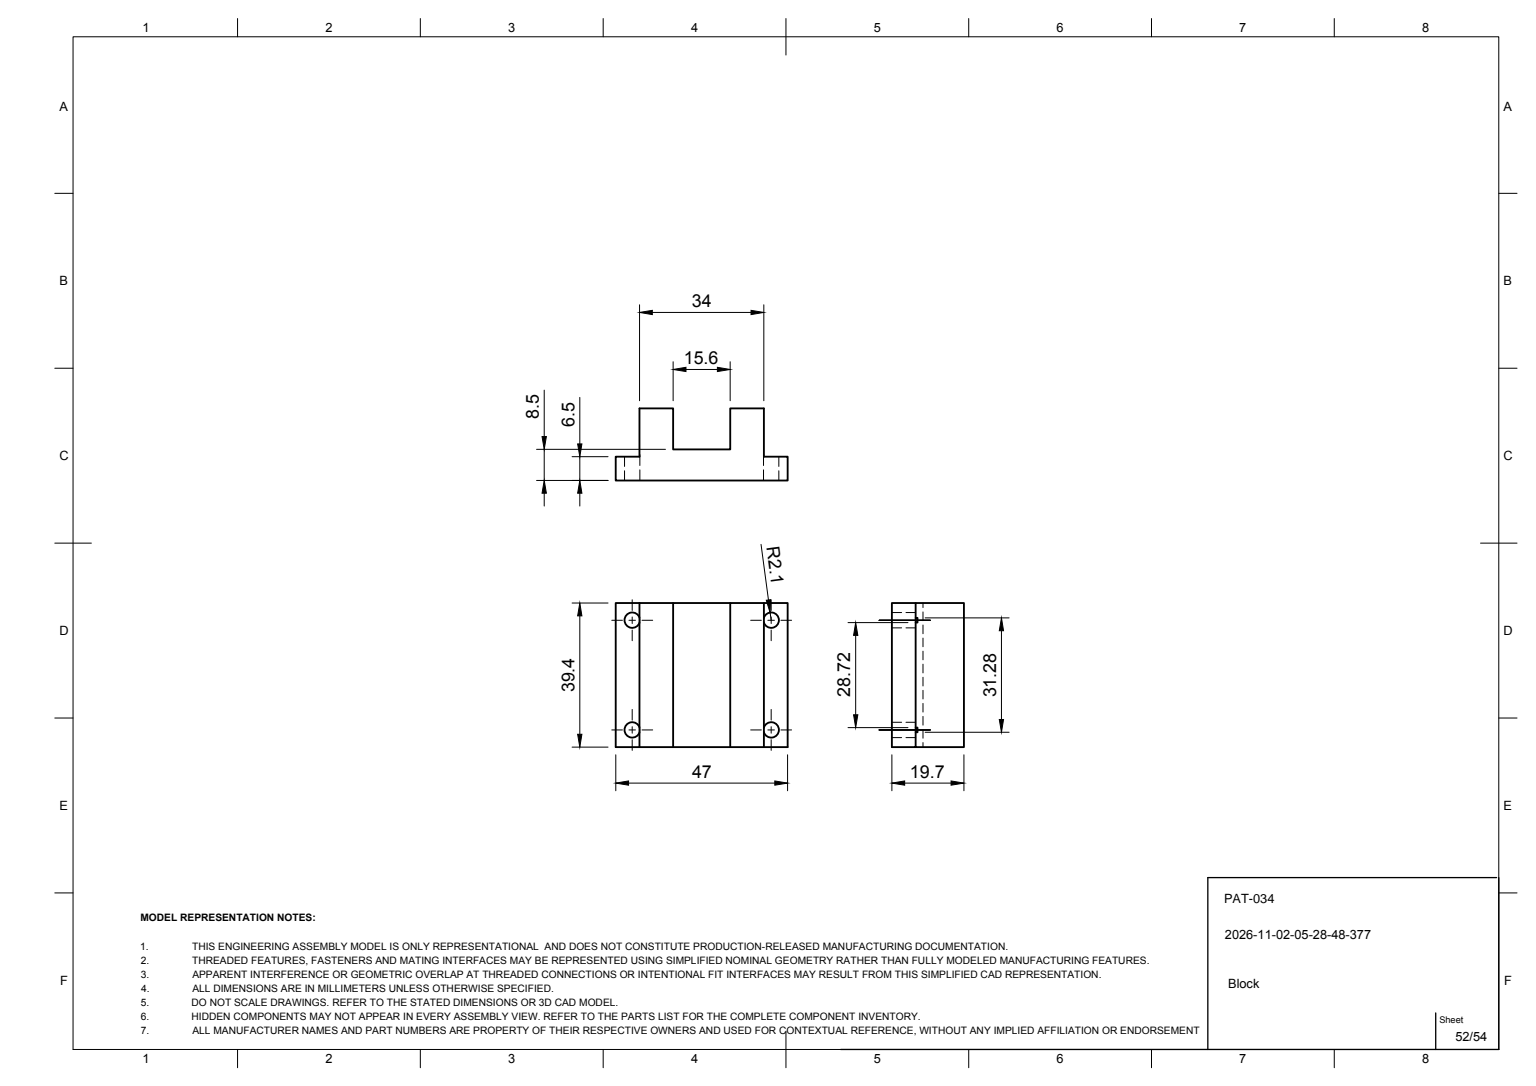
ISO-10303-21;
HEADER;
/* Generated by software containing ST-Developer
 * from STEP Tools, Inc. (www.steptools.com) 
 */

FILE_DESCRIPTION(
/* description */ ('Fatigue rig crank-slider'),
/* implementation_level */ '2;1');

FILE_NAME(
/* name */ 'Block.step',
/* time_stamp */ '2026-10-28T03:24:50-07:00',
/* author */ (''),
/* organization */ (''),
/* preprocessor_version */ 'ST-DEVELOPER v20.2',
/* originating_system */ 'Autodesk Translation Framework v15.17.0.0',
/* authorisation */ '');

FILE_SCHEMA (('AUTOMOTIVE_DESIGN { 1 0 10303 214 3 1 1 }'));
ENDSEC;

DATA;
#10=MECHANICAL_DESIGN_GEOMETRIC_PRESENTATION_REPRESENTATION('',(#639),#16911);
#530=SHAPE_REPRESENTATION_RELATIONSHIP('SRR','None',#17175,#580);
#580=ADVANCED_BREP_SHAPE_REPRESENTATION('',(#696),#16904);
#639=STYLED_ITEM('',(#17466),#696);
#696=MANIFOLD_SOLID_BREP('Body1',#8932);
#888=FACE_BOUND('',#2369,.T.);
#889=FACE_BOUND('',#2370,.T.);
#890=FACE_BOUND('',#2371,.T.);
#891=FACE_BOUND('',#2372,.T.);
#1144=PLANE('',#10343);
#1145=PLANE('',#10349);
#1146=PLANE('',#10355);
#1147=PLANE('',#10361);
#1148=PLANE('',#10367);
#1149=PLANE('',#10368);
#1150=PLANE('',#10369);
#1151=PLANE('',#10370);
#1152=PLANE('',#10371);
#1153=PLANE('',#10372);
#1154=PLANE('',#10373);
#1155=PLANE('',#10374);
#1156=PLANE('',#10375);
#1157=PLANE('',#10376);
#1158=PLANE('',#10377);
#1159=PLANE('',#10378);
#1160=PLANE('',#10379);
#1161=PLANE('',#10380);
#1644=FACE_OUTER_BOUND('',#2355,.T.);
#1645=FACE_OUTER_BOUND('',#2356,.T.);
#1646=FACE_OUTER_BOUND('',#2357,.T.);
#1647=FACE_OUTER_BOUND('',#2358,.T.);
#1648=FACE_OUTER_BOUND('',#2359,.T.);
#1649=FACE_OUTER_BOUND('',#2360,.T.);
#1650=FACE_OUTER_BOUND('',#2361,.T.);
#1651=FACE_OUTER_BOUND('',#2362,.T.);
#1652=FACE_OUTER_BOUND('',#2363,.T.);
#1653=FACE_OUTER_BOUND('',#2364,.T.);
#1654=FACE_OUTER_BOUND('',#2365,.T.);
#1655=FACE_OUTER_BOUND('',#2366,.T.);
#1656=FACE_OUTER_BOUND('',#2367,.T.);
#1657=FACE_OUTER_BOUND('',#2368,.T.);
#1658=FACE_OUTER_BOUND('',#2373,.T.);
#1659=FACE_OUTER_BOUND('',#2374,.T.);
#1660=FACE_OUTER_BOUND('',#2375,.T.);
#1661=FACE_OUTER_BOUND('',#2376,.T.);
#1662=FACE_OUTER_BOUND('',#2377,.T.);
#1663=FACE_OUTER_BOUND('',#2378,.T.);
#1664=FACE_OUTER_BOUND('',#2379,.T.);
#1665=FACE_OUTER_BOUND('',#2380,.T.);
#2355=EDGE_LOOP('',(#7756,#7757));
#2356=EDGE_LOOP('',(#7758,#7759,#7760,#7761,#7762,#7763,#7764,#7765));
#2357=EDGE_LOOP('',(#7766,#7767));
#2358=EDGE_LOOP('',(#7768,#7769,#7770,#7771,#7772,#7773,#7774,#7775));
#2359=EDGE_LOOP('',(#7776,#7777));
#2360=EDGE_LOOP('',(#7778,#7779,#7780,#7781,#7782,#7783,#7784,#7785));
#2361=EDGE_LOOP('',(#7786,#7787));
#2362=EDGE_LOOP('',(#7788,#7789,#7790,#7791,#7792,#7793,#7794,#7795));
#2363=EDGE_LOOP('',(#7796,#7797,#7798,#7799,#7800,#7801,#7802,#7803,#7804,
#7805,#7806,#7807));
#2364=EDGE_LOOP('',(#7808,#7809,#7810,#7811,#7812,#7813,#7814,#7815,#7816,
#7817,#7818,#7819));
#2365=EDGE_LOOP('',(#7820,#7821,#7822,#7823,#7824,#7825,#7826,#7827,#7828,
#7829,#7830,#7831));
#2366=EDGE_LOOP('',(#7832,#7833,#7834,#7835,#7836,#7837,#7838,#7839,#7840,
#7841));
#2367=EDGE_LOOP('',(#7842,#7843,#7844,#7845));
#2368=EDGE_LOOP('',(#7846,#7847,#7848,#7849));
#2369=EDGE_LOOP('',(#7850));
#2370=EDGE_LOOP('',(#7851));
#2371=EDGE_LOOP('',(#7852));
#2372=EDGE_LOOP('',(#7853));
#2373=EDGE_LOOP('',(#7854,#7855,#7856,#7857));
#2374=EDGE_LOOP('',(#7858,#7859,#7860,#7861,#7862,#7863,#7864,#7865,#7866,
#7867));
#2375=EDGE_LOOP('',(#7868,#7869,#7870,#7871));
#2376=EDGE_LOOP('',(#7872,#7873,#7874,#7875));
#2377=EDGE_LOOP('',(#7876,#7877,#7878,#7879));
#2378=EDGE_LOOP('',(#7880,#7881,#7882,#7883));
#2379=EDGE_LOOP('',(#7884,#7885,#7886,#7887));
#2380=EDGE_LOOP('',(#7888,#7889,#7890,#7891,#7892,#7893,#7894,#7895,#7896,
#7897,#7898,#7899));
#2929=LINE('',#16254,#3575);
#2930=LINE('',#16258,#3576);
#2931=LINE('',#16262,#3577);
#2932=LINE('',#16266,#3578);
#2933=LINE('',#16270,#3579);
#2934=LINE('',#16274,#3580);
#2935=LINE('',#16278,#3581);
#2936=LINE('',#16282,#3582);
#2937=LINE('',#16286,#3583);
#2938=LINE('',#16290,#3584);
#2939=LINE('',#16294,#3585);
#2940=LINE('',#16298,#3586);
#2941=LINE('',#16302,#3587);
#2942=LINE('',#16306,#3588);
#2943=LINE('',#16310,#3589);
#2944=LINE('',#16314,#3590);
#2945=LINE('',#16316,#3591);
#2946=LINE('',#16318,#3592);
#2947=LINE('',#16320,#3593);
#2948=LINE('',#16322,#3594);
#2949=LINE('',#16324,#3595);
#2950=LINE('',#16325,#3596);
#2951=LINE('',#16327,#3597);
#2952=LINE('',#16329,#3598);
#2953=LINE('',#16331,#3599);
#2954=LINE('',#16333,#3600);
#2955=LINE('',#16335,#3601);
#2956=LINE('',#16336,#3602);
#2957=LINE('',#16339,#3603);
#2958=LINE('',#16341,#3604);
#2959=LINE('',#16343,#3605);
#2960=LINE('',#16345,#3606);
#2961=LINE('',#16346,#3607);
#2962=LINE('',#16348,#3608);
#2963=LINE('',#16350,#3609);
#2964=LINE('',#16352,#3610);
#2965=LINE('',#16354,#3611);
#2966=LINE('',#16355,#3612);
#2967=LINE('',#16358,#3613);
#2968=LINE('',#16359,#3614);
#2969=LINE('',#16362,#3615);
#2970=LINE('',#16363,#3616);
#2971=LINE('',#16366,#3617);
#2972=LINE('',#16367,#3618);
#2973=LINE('',#16370,#3619);
#2974=LINE('',#16371,#3620);
#2975=LINE('',#16373,#3621);
#2976=LINE('',#16376,#3622);
#2977=LINE('',#16377,#3623);
#2978=LINE('',#16380,#3624);
#2979=LINE('',#16381,#3625);
#2980=LINE('',#16384,#3626);
#2981=LINE('',#16385,#3627);
#2982=LINE('',#16388,#3628);
#2983=LINE('',#16389,#3629);
#2984=LINE('',#16391,#3630);
#3575=VECTOR('',#12737,1.);
#3576=VECTOR('',#12742,1.);
#3577=VECTOR('',#12745,0.21);
#3578=VECTOR('',#12750,1.);
#3579=VECTOR('',#12753,1.);
#3580=VECTOR('',#12758,1.);
#3581=VECTOR('',#12761,0.21);
#3582=VECTOR('',#12766,1.);
#3583=VECTOR('',#12769,1.);
#3584=VECTOR('',#12774,1.);
#3585=VECTOR('',#12777,0.21);
#3586=VECTOR('',#12782,1.);
#3587=VECTOR('',#12785,1.);
#3588=VECTOR('',#12790,1.);
#3589=VECTOR('',#12793,0.21);
#3590=VECTOR('',#12798,1.);
#3591=VECTOR('',#12801,1.);
#3592=VECTOR('',#12802,1.);
#3593=VECTOR('',#12803,1.);
#3594=VECTOR('',#12804,1.);
#3595=VECTOR('',#12805,1.);
#3596=VECTOR('',#12806,1.);
#3597=VECTOR('',#12809,1.);
#3598=VECTOR('',#12810,1.);
#3599=VECTOR('',#12811,1.);
#3600=VECTOR('',#12812,1.);
#3601=VECTOR('',#12813,1.);
#3602=VECTOR('',#12814,1.);
#3603=VECTOR('',#12817,1.);
#3604=VECTOR('',#12818,1.);
#3605=VECTOR('',#12819,1.);
#3606=VECTOR('',#12820,1.);
#3607=VECTOR('',#12821,1.);
#3608=VECTOR('',#12822,1.);
#3609=VECTOR('',#12823,1.);
#3610=VECTOR('',#12824,1.);
#3611=VECTOR('',#12825,1.);
#3612=VECTOR('',#12826,1.);
#3613=VECTOR('',#12829,1.);
#3614=VECTOR('',#12830,1.);
#3615=VECTOR('',#12833,1.);
#3616=VECTOR('',#12834,1.);
#3617=VECTOR('',#12837,1.);
#3618=VECTOR('',#12838,1.);
#3619=VECTOR('',#12841,1.);
#3620=VECTOR('',#12842,1.);
#3621=VECTOR('',#12845,1.);
#3622=VECTOR('',#12848,1.);
#3623=VECTOR('',#12849,1.);
#3624=VECTOR('',#12852,1.);
#3625=VECTOR('',#12853,1.);
#3626=VECTOR('',#12856,1.);
#3627=VECTOR('',#12857,1.);
#3628=VECTOR('',#12860,1.);
#3629=VECTOR('',#12861,1.);
#3630=VECTOR('',#12864,1.);
#4109=CIRCLE('',#10344,0.21);
#4110=CIRCLE('',#10346,0.21);
#4111=CIRCLE('',#10347,0.21);
#4112=CIRCLE('',#10348,0.21);
#4113=CIRCLE('',#10350,0.21);
#4114=CIRCLE('',#10352,0.21);
#4115=CIRCLE('',#10353,0.21);
#4116=CIRCLE('',#10354,0.21);
#4117=CIRCLE('',#10356,0.21);
#4118=CIRCLE('',#10358,0.21);
#4119=CIRCLE('',#10359,0.21);
#4120=CIRCLE('',#10360,0.21);
#4121=CIRCLE('',#10362,0.21);
#4122=CIRCLE('',#10364,0.21);
#4123=CIRCLE('',#10365,0.21);
#4124=CIRCLE('',#10366,0.21);
#4753=VERTEX_POINT('',#16252);
#4754=VERTEX_POINT('',#16253);
#4755=VERTEX_POINT('',#16257);
#4756=VERTEX_POINT('',#16259);
#4757=VERTEX_POINT('',#16261);
#4758=VERTEX_POINT('',#16264);
#4759=VERTEX_POINT('',#16268);
#4760=VERTEX_POINT('',#16269);
#4761=VERTEX_POINT('',#16273);
#4762=VERTEX_POINT('',#16275);
#4763=VERTEX_POINT('',#16277);
#4764=VERTEX_POINT('',#16280);
#4765=VERTEX_POINT('',#16284);
#4766=VERTEX_POINT('',#16285);
#4767=VERTEX_POINT('',#16289);
#4768=VERTEX_POINT('',#16291);
#4769=VERTEX_POINT('',#16293);
#4770=VERTEX_POINT('',#16296);
#4771=VERTEX_POINT('',#16300);
#4772=VERTEX_POINT('',#16301);
#4773=VERTEX_POINT('',#16305);
#4774=VERTEX_POINT('',#16307);
#4775=VERTEX_POINT('',#16309);
#4776=VERTEX_POINT('',#16312);
#4777=VERTEX_POINT('',#16317);
#4778=VERTEX_POINT('',#16319);
#4779=VERTEX_POINT('',#16321);
#4780=VERTEX_POINT('',#16323);
#4781=VERTEX_POINT('',#16328);
#4782=VERTEX_POINT('',#16330);
#4783=VERTEX_POINT('',#16332);
#4784=VERTEX_POINT('',#16334);
#4785=VERTEX_POINT('',#16338);
#4786=VERTEX_POINT('',#16340);
#4787=VERTEX_POINT('',#16342);
#4788=VERTEX_POINT('',#16344);
#4789=VERTEX_POINT('',#16347);
#4790=VERTEX_POINT('',#16349);
#4791=VERTEX_POINT('',#16351);
#4792=VERTEX_POINT('',#16353);
#4793=VERTEX_POINT('',#16357);
#4794=VERTEX_POINT('',#16361);
#4795=VERTEX_POINT('',#16365);
#4796=VERTEX_POINT('',#16369);
#4797=VERTEX_POINT('',#16375);
#4798=VERTEX_POINT('',#16379);
#4799=VERTEX_POINT('',#16383);
#4800=VERTEX_POINT('',#16387);
#5776=EDGE_CURVE('',#4753,#4754,#2929,.T.);
#5777=EDGE_CURVE('',#4753,#4754,#4109,.T.);
#5778=EDGE_CURVE('',#4755,#4753,#2930,.T.);
#5779=EDGE_CURVE('',#4756,#4755,#4110,.T.);
#5780=EDGE_CURVE('',#4756,#4757,#2931,.T.);
#5781=EDGE_CURVE('',#4757,#4757,#4111,.T.);
#5782=EDGE_CURVE('',#4758,#4756,#4112,.T.);
#5783=EDGE_CURVE('',#4754,#4758,#2932,.T.);
#5784=EDGE_CURVE('',#4759,#4760,#2933,.T.);
#5785=EDGE_CURVE('',#4759,#4760,#4113,.T.);
#5786=EDGE_CURVE('',#4761,#4759,#2934,.T.);
#5787=EDGE_CURVE('',#4762,#4761,#4114,.T.);
#5788=EDGE_CURVE('',#4762,#4763,#2935,.T.);
#5789=EDGE_CURVE('',#4763,#4763,#4115,.T.);
#5790=EDGE_CURVE('',#4764,#4762,#4116,.T.);
#5791=EDGE_CURVE('',#4760,#4764,#2936,.T.);
#5792=EDGE_CURVE('',#4765,#4766,#2937,.T.);
#5793=EDGE_CURVE('',#4765,#4766,#4117,.T.);
#5794=EDGE_CURVE('',#4767,#4765,#2938,.T.);
#5795=EDGE_CURVE('',#4768,#4767,#4118,.T.);
#5796=EDGE_CURVE('',#4768,#4769,#2939,.T.);
#5797=EDGE_CURVE('',#4769,#4769,#4119,.T.);
#5798=EDGE_CURVE('',#4770,#4768,#4120,.T.);
#5799=EDGE_CURVE('',#4766,#4770,#2940,.T.);
#5800=EDGE_CURVE('',#4771,#4772,#2941,.T.);
#5801=EDGE_CURVE('',#4771,#4772,#4121,.T.);
#5802=EDGE_CURVE('',#4773,#4771,#2942,.T.);
#5803=EDGE_CURVE('',#4774,#4773,#4122,.T.);
#5804=EDGE_CURVE('',#4774,#4775,#2943,.T.);
#5805=EDGE_CURVE('',#4775,#4775,#4123,.T.);
#5806=EDGE_CURVE('',#4776,#4774,#4124,.T.);
#5807=EDGE_CURVE('',#4772,#4776,#2944,.T.);
#5808=EDGE_CURVE('',#4758,#4767,#2945,.T.);
#5809=EDGE_CURVE('',#4770,#4777,#2946,.T.);
#5810=EDGE_CURVE('',#4778,#4777,#2947,.T.);
#5811=EDGE_CURVE('',#4778,#4779,#2948,.T.);
#5812=EDGE_CURVE('',#4780,#4779,#2949,.T.);
#5813=EDGE_CURVE('',#4780,#4755,#2950,.T.);
#5814=EDGE_CURVE('',#4764,#4773,#2951,.T.);
#5815=EDGE_CURVE('',#4776,#4781,#2952,.T.);
#5816=EDGE_CURVE('',#4782,#4781,#2953,.T.);
#5817=EDGE_CURVE('',#4783,#4782,#2954,.T.);
#5818=EDGE_CURVE('',#4784,#4783,#2955,.T.);
#5819=EDGE_CURVE('',#4784,#4761,#2956,.T.);
#5820=EDGE_CURVE('',#4777,#4785,#2957,.T.);
#5821=EDGE_CURVE('',#4785,#4786,#2958,.T.);
#5822=EDGE_CURVE('',#4786,#4787,#2959,.T.);
#5823=EDGE_CURVE('',#4787,#4788,#2960,.T.);
#5824=EDGE_CURVE('',#4788,#4784,#2961,.T.);
#5825=EDGE_CURVE('',#4783,#4789,#2962,.T.);
#5826=EDGE_CURVE('',#4789,#4790,#2963,.T.);
#5827=EDGE_CURVE('',#4790,#4791,#2964,.T.);
#5828=EDGE_CURVE('',#4791,#4792,#2965,.T.);
#5829=EDGE_CURVE('',#4792,#4778,#2966,.T.);
#5830=EDGE_CURVE('',#4793,#4780,#2967,.T.);
#5831=EDGE_CURVE('',#4785,#4793,#2968,.T.);
#5832=EDGE_CURVE('',#4794,#4793,#2969,.T.);
#5833=EDGE_CURVE('',#4786,#4794,#2970,.T.);
#5834=EDGE_CURVE('',#4795,#4794,#2971,.T.);
#5835=EDGE_CURVE('',#4787,#4795,#2972,.T.);
#5836=EDGE_CURVE('',#4796,#4795,#2973,.T.);
#5837=EDGE_CURVE('',#4788,#4796,#2974,.T.);
#5838=EDGE_CURVE('',#4781,#4796,#2975,.T.);
#5839=EDGE_CURVE('',#4797,#4782,#2976,.T.);
#5840=EDGE_CURVE('',#4789,#4797,#2977,.T.);
#5841=EDGE_CURVE('',#4798,#4797,#2978,.T.);
#5842=EDGE_CURVE('',#4790,#4798,#2979,.T.);
#5843=EDGE_CURVE('',#4799,#4798,#2980,.T.);
#5844=EDGE_CURVE('',#4791,#4799,#2981,.T.);
#5845=EDGE_CURVE('',#4800,#4799,#2982,.T.);
#5846=EDGE_CURVE('',#4792,#4800,#2983,.T.);
#5847=EDGE_CURVE('',#4779,#4800,#2984,.T.);
#7756=ORIENTED_EDGE('',*,*,#5776,.F.);
#7757=ORIENTED_EDGE('',*,*,#5777,.T.);
#7758=ORIENTED_EDGE('',*,*,#5778,.F.);
#7759=ORIENTED_EDGE('',*,*,#5779,.F.);
#7760=ORIENTED_EDGE('',*,*,#5780,.T.);
#7761=ORIENTED_EDGE('',*,*,#5781,.F.);
#7762=ORIENTED_EDGE('',*,*,#5780,.F.);
#7763=ORIENTED_EDGE('',*,*,#5782,.F.);
#7764=ORIENTED_EDGE('',*,*,#5783,.F.);
#7765=ORIENTED_EDGE('',*,*,#5777,.F.);
#7766=ORIENTED_EDGE('',*,*,#5784,.F.);
#7767=ORIENTED_EDGE('',*,*,#5785,.T.);
#7768=ORIENTED_EDGE('',*,*,#5786,.F.);
#7769=ORIENTED_EDGE('',*,*,#5787,.F.);
#7770=ORIENTED_EDGE('',*,*,#5788,.T.);
#7771=ORIENTED_EDGE('',*,*,#5789,.F.);
#7772=ORIENTED_EDGE('',*,*,#5788,.F.);
#7773=ORIENTED_EDGE('',*,*,#5790,.F.);
#7774=ORIENTED_EDGE('',*,*,#5791,.F.);
#7775=ORIENTED_EDGE('',*,*,#5785,.F.);
#7776=ORIENTED_EDGE('',*,*,#5792,.F.);
#7777=ORIENTED_EDGE('',*,*,#5793,.T.);
#7778=ORIENTED_EDGE('',*,*,#5794,.F.);
#7779=ORIENTED_EDGE('',*,*,#5795,.F.);
#7780=ORIENTED_EDGE('',*,*,#5796,.T.);
#7781=ORIENTED_EDGE('',*,*,#5797,.F.);
#7782=ORIENTED_EDGE('',*,*,#5796,.F.);
#7783=ORIENTED_EDGE('',*,*,#5798,.F.);
#7784=ORIENTED_EDGE('',*,*,#5799,.F.);
#7785=ORIENTED_EDGE('',*,*,#5793,.F.);
#7786=ORIENTED_EDGE('',*,*,#5800,.F.);
#7787=ORIENTED_EDGE('',*,*,#5801,.T.);
#7788=ORIENTED_EDGE('',*,*,#5802,.F.);
#7789=ORIENTED_EDGE('',*,*,#5803,.F.);
#7790=ORIENTED_EDGE('',*,*,#5804,.T.);
#7791=ORIENTED_EDGE('',*,*,#5805,.F.);
#7792=ORIENTED_EDGE('',*,*,#5804,.F.);
#7793=ORIENTED_EDGE('',*,*,#5806,.F.);
#7794=ORIENTED_EDGE('',*,*,#5807,.F.);
#7795=ORIENTED_EDGE('',*,*,#5801,.F.);
#7796=ORIENTED_EDGE('',*,*,#5778,.T.);
#7797=ORIENTED_EDGE('',*,*,#5776,.T.);
#7798=ORIENTED_EDGE('',*,*,#5783,.T.);
#7799=ORIENTED_EDGE('',*,*,#5808,.T.);
#7800=ORIENTED_EDGE('',*,*,#5794,.T.);
#7801=ORIENTED_EDGE('',*,*,#5792,.T.);
#7802=ORIENTED_EDGE('',*,*,#5799,.T.);
#7803=ORIENTED_EDGE('',*,*,#5809,.T.);
#7804=ORIENTED_EDGE('',*,*,#5810,.F.);
#7805=ORIENTED_EDGE('',*,*,#5811,.T.);
#7806=ORIENTED_EDGE('',*,*,#5812,.F.);
#7807=ORIENTED_EDGE('',*,*,#5813,.T.);
#7808=ORIENTED_EDGE('',*,*,#5786,.T.);
#7809=ORIENTED_EDGE('',*,*,#5784,.T.);
#7810=ORIENTED_EDGE('',*,*,#5791,.T.);
#7811=ORIENTED_EDGE('',*,*,#5814,.T.);
#7812=ORIENTED_EDGE('',*,*,#5802,.T.);
#7813=ORIENTED_EDGE('',*,*,#5800,.T.);
#7814=ORIENTED_EDGE('',*,*,#5807,.T.);
#7815=ORIENTED_EDGE('',*,*,#5815,.T.);
#7816=ORIENTED_EDGE('',*,*,#5816,.F.);
#7817=ORIENTED_EDGE('',*,*,#5817,.F.);
#7818=ORIENTED_EDGE('',*,*,#5818,.F.);
#7819=ORIENTED_EDGE('',*,*,#5819,.T.);
#7820=ORIENTED_EDGE('',*,*,#5810,.T.);
#7821=ORIENTED_EDGE('',*,*,#5820,.T.);
#7822=ORIENTED_EDGE('',*,*,#5821,.T.);
#7823=ORIENTED_EDGE('',*,*,#5822,.T.);
#7824=ORIENTED_EDGE('',*,*,#5823,.T.);
#7825=ORIENTED_EDGE('',*,*,#5824,.T.);
#7826=ORIENTED_EDGE('',*,*,#5818,.T.);
#7827=ORIENTED_EDGE('',*,*,#5825,.T.);
#7828=ORIENTED_EDGE('',*,*,#5826,.T.);
#7829=ORIENTED_EDGE('',*,*,#5827,.T.);
#7830=ORIENTED_EDGE('',*,*,#5828,.T.);
#7831=ORIENTED_EDGE('',*,*,#5829,.T.);
#7832=ORIENTED_EDGE('',*,*,#5782,.T.);
#7833=ORIENTED_EDGE('',*,*,#5779,.T.);
#7834=ORIENTED_EDGE('',*,*,#5813,.F.);
#7835=ORIENTED_EDGE('',*,*,#5830,.F.);
#7836=ORIENTED_EDGE('',*,*,#5831,.F.);
#7837=ORIENTED_EDGE('',*,*,#5820,.F.);
#7838=ORIENTED_EDGE('',*,*,#5809,.F.);
#7839=ORIENTED_EDGE('',*,*,#5798,.T.);
#7840=ORIENTED_EDGE('',*,*,#5795,.T.);
#7841=ORIENTED_EDGE('',*,*,#5808,.F.);
#7842=ORIENTED_EDGE('',*,*,#5831,.T.);
#7843=ORIENTED_EDGE('',*,*,#5832,.F.);
#7844=ORIENTED_EDGE('',*,*,#5833,.F.);
#7845=ORIENTED_EDGE('',*,*,#5821,.F.);
#7846=ORIENTED_EDGE('',*,*,#5833,.T.);
#7847=ORIENTED_EDGE('',*,*,#5834,.F.);
#7848=ORIENTED_EDGE('',*,*,#5835,.F.);
#7849=ORIENTED_EDGE('',*,*,#5822,.F.);
#7850=ORIENTED_EDGE('',*,*,#5781,.T.);
#7851=ORIENTED_EDGE('',*,*,#5789,.T.);
#7852=ORIENTED_EDGE('',*,*,#5797,.T.);
#7853=ORIENTED_EDGE('',*,*,#5805,.T.);
#7854=ORIENTED_EDGE('',*,*,#5835,.T.);
#7855=ORIENTED_EDGE('',*,*,#5836,.F.);
#7856=ORIENTED_EDGE('',*,*,#5837,.F.);
#7857=ORIENTED_EDGE('',*,*,#5823,.F.);
#7858=ORIENTED_EDGE('',*,*,#5790,.T.);
#7859=ORIENTED_EDGE('',*,*,#5787,.T.);
#7860=ORIENTED_EDGE('',*,*,#5819,.F.);
#7861=ORIENTED_EDGE('',*,*,#5824,.F.);
#7862=ORIENTED_EDGE('',*,*,#5837,.T.);
#7863=ORIENTED_EDGE('',*,*,#5838,.F.);
#7864=ORIENTED_EDGE('',*,*,#5815,.F.);
#7865=ORIENTED_EDGE('',*,*,#5806,.T.);
#7866=ORIENTED_EDGE('',*,*,#5803,.T.);
#7867=ORIENTED_EDGE('',*,*,#5814,.F.);
#7868=ORIENTED_EDGE('',*,*,#5817,.T.);
#7869=ORIENTED_EDGE('',*,*,#5839,.F.);
#7870=ORIENTED_EDGE('',*,*,#5840,.F.);
#7871=ORIENTED_EDGE('',*,*,#5825,.F.);
#7872=ORIENTED_EDGE('',*,*,#5840,.T.);
#7873=ORIENTED_EDGE('',*,*,#5841,.F.);
#7874=ORIENTED_EDGE('',*,*,#5842,.F.);
#7875=ORIENTED_EDGE('',*,*,#5826,.F.);
#7876=ORIENTED_EDGE('',*,*,#5842,.T.);
#7877=ORIENTED_EDGE('',*,*,#5843,.F.);
#7878=ORIENTED_EDGE('',*,*,#5844,.F.);
#7879=ORIENTED_EDGE('',*,*,#5827,.F.);
#7880=ORIENTED_EDGE('',*,*,#5844,.T.);
#7881=ORIENTED_EDGE('',*,*,#5845,.F.);
#7882=ORIENTED_EDGE('',*,*,#5846,.F.);
#7883=ORIENTED_EDGE('',*,*,#5828,.F.);
#7884=ORIENTED_EDGE('',*,*,#5846,.T.);
#7885=ORIENTED_EDGE('',*,*,#5847,.F.);
#7886=ORIENTED_EDGE('',*,*,#5811,.F.);
#7887=ORIENTED_EDGE('',*,*,#5829,.F.);
#7888=ORIENTED_EDGE('',*,*,#5812,.T.);
#7889=ORIENTED_EDGE('',*,*,#5847,.T.);
#7890=ORIENTED_EDGE('',*,*,#5845,.T.);
#7891=ORIENTED_EDGE('',*,*,#5843,.T.);
#7892=ORIENTED_EDGE('',*,*,#5841,.T.);
#7893=ORIENTED_EDGE('',*,*,#5839,.T.);
#7894=ORIENTED_EDGE('',*,*,#5816,.T.);
#7895=ORIENTED_EDGE('',*,*,#5838,.T.);
#7896=ORIENTED_EDGE('',*,*,#5836,.T.);
#7897=ORIENTED_EDGE('',*,*,#5834,.T.);
#7898=ORIENTED_EDGE('',*,*,#5832,.T.);
#7899=ORIENTED_EDGE('',*,*,#5830,.T.);
#8343=CYLINDRICAL_SURFACE('',#10345,0.21);
#8344=CYLINDRICAL_SURFACE('',#10351,0.21);
#8345=CYLINDRICAL_SURFACE('',#10357,0.21);
#8346=CYLINDRICAL_SURFACE('',#10363,0.21);
#8782=ADVANCED_FACE('',(#1644),#1144,.T.);
#8783=ADVANCED_FACE('',(#1645),#8343,.F.);
#8784=ADVANCED_FACE('',(#1646),#1145,.T.);
#8785=ADVANCED_FACE('',(#1647),#8344,.F.);
#8786=ADVANCED_FACE('',(#1648),#1146,.T.);
#8787=ADVANCED_FACE('',(#1649),#8345,.F.);
#8788=ADVANCED_FACE('',(#1650),#1147,.T.);
#8789=ADVANCED_FACE('',(#1651),#8346,.F.);
#8790=ADVANCED_FACE('',(#1652),#1148,.T.);
#8791=ADVANCED_FACE('',(#1653),#1149,.T.);
#8792=ADVANCED_FACE('',(#1654),#1150,.T.);
#8793=ADVANCED_FACE('',(#1655),#1151,.T.);
#8794=ADVANCED_FACE('',(#1656),#1152,.T.);
#8795=ADVANCED_FACE('',(#1657,#888,#889,#890,#891),#1153,.T.);
#8796=ADVANCED_FACE('',(#1658),#1154,.T.);
#8797=ADVANCED_FACE('',(#1659),#1155,.T.);
#8798=ADVANCED_FACE('',(#1660),#1156,.T.);
#8799=ADVANCED_FACE('',(#1661),#1157,.T.);
#8800=ADVANCED_FACE('',(#1662),#1158,.T.);
#8801=ADVANCED_FACE('',(#1663),#1159,.T.);
#8802=ADVANCED_FACE('',(#1664),#1160,.T.);
#8803=ADVANCED_FACE('',(#1665),#1161,.T.);
#8932=CLOSED_SHELL('',(#8782,#8783,#8784,#8785,#8786,#8787,#8788,#8789,
#8790,#8791,#8792,#8793,#8794,#8795,#8796,#8797,#8798,#8799,#8800,#8801,
#8802,#8803));
#10342=AXIS2_PLACEMENT_3D('',#16250,#12733,#12734);
#10343=AXIS2_PLACEMENT_3D('',#16251,#12735,#12736);
#10344=AXIS2_PLACEMENT_3D('',#16255,#12738,#12739);
#10345=AXIS2_PLACEMENT_3D('',#16256,#12740,#12741);
#10346=AXIS2_PLACEMENT_3D('',#16260,#12743,#12744);
#10347=AXIS2_PLACEMENT_3D('',#16263,#12746,#12747);
#10348=AXIS2_PLACEMENT_3D('',#16265,#12748,#12749);
#10349=AXIS2_PLACEMENT_3D('',#16267,#12751,#12752);
#10350=AXIS2_PLACEMENT_3D('',#16271,#12754,#12755);
#10351=AXIS2_PLACEMENT_3D('',#16272,#12756,#12757);
#10352=AXIS2_PLACEMENT_3D('',#16276,#12759,#12760);
#10353=AXIS2_PLACEMENT_3D('',#16279,#12762,#12763);
#10354=AXIS2_PLACEMENT_3D('',#16281,#12764,#12765);
#10355=AXIS2_PLACEMENT_3D('',#16283,#12767,#12768);
#10356=AXIS2_PLACEMENT_3D('',#16287,#12770,#12771);
#10357=AXIS2_PLACEMENT_3D('',#16288,#12772,#12773);
#10358=AXIS2_PLACEMENT_3D('',#16292,#12775,#12776);
#10359=AXIS2_PLACEMENT_3D('',#16295,#12778,#12779);
#10360=AXIS2_PLACEMENT_3D('',#16297,#12780,#12781);
#10361=AXIS2_PLACEMENT_3D('',#16299,#12783,#12784);
#10362=AXIS2_PLACEMENT_3D('',#16303,#12786,#12787);
#10363=AXIS2_PLACEMENT_3D('',#16304,#12788,#12789);
#10364=AXIS2_PLACEMENT_3D('',#16308,#12791,#12792);
#10365=AXIS2_PLACEMENT_3D('',#16311,#12794,#12795);
#10366=AXIS2_PLACEMENT_3D('',#16313,#12796,#12797);
#10367=AXIS2_PLACEMENT_3D('',#16315,#12799,#12800);
#10368=AXIS2_PLACEMENT_3D('',#16326,#12807,#12808);
#10369=AXIS2_PLACEMENT_3D('',#16337,#12815,#12816);
#10370=AXIS2_PLACEMENT_3D('',#16356,#12827,#12828);
#10371=AXIS2_PLACEMENT_3D('',#16360,#12831,#12832);
#10372=AXIS2_PLACEMENT_3D('',#16364,#12835,#12836);
#10373=AXIS2_PLACEMENT_3D('',#16368,#12839,#12840);
#10374=AXIS2_PLACEMENT_3D('',#16372,#12843,#12844);
#10375=AXIS2_PLACEMENT_3D('',#16374,#12846,#12847);
#10376=AXIS2_PLACEMENT_3D('',#16378,#12850,#12851);
#10377=AXIS2_PLACEMENT_3D('',#16382,#12854,#12855);
#10378=AXIS2_PLACEMENT_3D('',#16386,#12858,#12859);
#10379=AXIS2_PLACEMENT_3D('',#16390,#12862,#12863);
#10380=AXIS2_PLACEMENT_3D('',#16392,#12865,#12866);
#12733=DIRECTION('axis',(0.,0.,1.));
#12734=DIRECTION('refdir',(1.,0.,0.));
#12735=DIRECTION('center_axis',(0.,0.,1.));
#12736=DIRECTION('ref_axis',(1.,0.,0.));
#12737=DIRECTION('',(-1.,0.,0.));
#12738=DIRECTION('center_axis',(0.,0.,1.));
#12739=DIRECTION('ref_axis',(1.,0.,0.));
#12740=DIRECTION('center_axis',(0.,0.,1.));
#12741=DIRECTION('ref_axis',(1.,0.,0.));
#12742=DIRECTION('',(0.,0.,-1.));
#12743=DIRECTION('center_axis',(0.,0.,1.));
#12744=DIRECTION('ref_axis',(1.,0.,0.));
#12745=DIRECTION('',(0.,0.,1.));
#12746=DIRECTION('center_axis',(0.,0.,-1.));
#12747=DIRECTION('ref_axis',(1.,0.,0.));
#12748=DIRECTION('center_axis',(0.,0.,1.));
#12749=DIRECTION('ref_axis',(1.,0.,0.));
#12750=DIRECTION('',(0.,0.,1.));
#12751=DIRECTION('center_axis',(0.,0.,1.));
#12752=DIRECTION('ref_axis',(1.,0.,0.));
#12753=DIRECTION('',(1.,0.,0.));
#12754=DIRECTION('center_axis',(0.,0.,1.));
#12755=DIRECTION('ref_axis',(1.,0.,0.));
#12756=DIRECTION('center_axis',(0.,0.,1.));
#12757=DIRECTION('ref_axis',(1.,0.,0.));
#12758=DIRECTION('',(0.,0.,-1.));
#12759=DIRECTION('center_axis',(0.,0.,1.));
#12760=DIRECTION('ref_axis',(1.,0.,0.));
#12761=DIRECTION('',(0.,0.,1.));
#12762=DIRECTION('center_axis',(0.,0.,-1.));
#12763=DIRECTION('ref_axis',(1.,0.,0.));
#12764=DIRECTION('center_axis',(0.,0.,1.));
#12765=DIRECTION('ref_axis',(1.,0.,0.));
#12766=DIRECTION('',(0.,0.,1.));
#12767=DIRECTION('center_axis',(0.,0.,1.));
#12768=DIRECTION('ref_axis',(1.,0.,0.));
#12769=DIRECTION('',(-1.,0.,0.));
#12770=DIRECTION('center_axis',(0.,0.,1.));
#12771=DIRECTION('ref_axis',(1.,0.,0.));
#12772=DIRECTION('center_axis',(0.,0.,1.));
#12773=DIRECTION('ref_axis',(1.,0.,0.));
#12774=DIRECTION('',(0.,0.,-1.));
#12775=DIRECTION('center_axis',(0.,0.,1.));
#12776=DIRECTION('ref_axis',(1.,0.,0.));
#12777=DIRECTION('',(0.,0.,1.));
#12778=DIRECTION('center_axis',(0.,0.,-1.));
#12779=DIRECTION('ref_axis',(1.,0.,0.));
#12780=DIRECTION('center_axis',(0.,0.,1.));
#12781=DIRECTION('ref_axis',(1.,0.,0.));
#12782=DIRECTION('',(0.,0.,1.));
#12783=DIRECTION('center_axis',(0.,0.,1.));
#12784=DIRECTION('ref_axis',(1.,0.,0.));
#12785=DIRECTION('',(1.,0.,0.));
#12786=DIRECTION('center_axis',(0.,0.,1.));
#12787=DIRECTION('ref_axis',(1.,0.,0.));
#12788=DIRECTION('center_axis',(0.,0.,1.));
#12789=DIRECTION('ref_axis',(1.,0.,0.));
#12790=DIRECTION('',(0.,0.,-1.));
#12791=DIRECTION('center_axis',(0.,0.,1.));
#12792=DIRECTION('ref_axis',(1.,0.,0.));
#12793=DIRECTION('',(0.,0.,1.));
#12794=DIRECTION('center_axis',(0.,0.,-1.));
#12795=DIRECTION('ref_axis',(1.,0.,0.));
#12796=DIRECTION('center_axis',(0.,0.,1.));
#12797=DIRECTION('ref_axis',(1.,0.,0.));
#12798=DIRECTION('',(0.,0.,1.));
#12799=DIRECTION('center_axis',(0.,-1.,0.));
#12800=DIRECTION('ref_axis',(0.,0.,-1.));
#12801=DIRECTION('',(-1.,0.,0.));
#12802=DIRECTION('',(-1.,0.,0.));
#12803=DIRECTION('',(0.,0.,1.));
#12804=DIRECTION('',(1.,0.,0.));
#12805=DIRECTION('',(0.,0.,-1.));
#12806=DIRECTION('',(-1.,0.,0.));
#12807=DIRECTION('center_axis',(0.,1.,0.));
#12808=DIRECTION('ref_axis',(0.,0.,1.));
#12809=DIRECTION('',(1.,0.,0.));
#12810=DIRECTION('',(1.,0.,0.));
#12811=DIRECTION('',(0.,0.,1.));
#12812=DIRECTION('',(1.,0.,0.));
#12813=DIRECTION('',(0.,0.,-1.));
#12814=DIRECTION('',(1.,0.,0.));
#12815=DIRECTION('center_axis',(-1.,0.,0.));
#12816=DIRECTION('ref_axis',(0.,0.,1.));
#12817=DIRECTION('',(0.,-1.,0.));
#12818=DIRECTION('',(0.,0.,1.));
#12819=DIRECTION('',(0.,1.,0.));
#12820=DIRECTION('',(0.,0.,-1.));
#12821=DIRECTION('',(0.,-1.,0.));
#12822=DIRECTION('',(0.,-1.,0.));
#12823=DIRECTION('',(0.,0.,1.));
#12824=DIRECTION('',(0.,-1.,0.));
#12825=DIRECTION('',(0.,0.,-1.));
#12826=DIRECTION('',(0.,-1.,0.));
#12827=DIRECTION('center_axis',(0.,0.,-1.));
#12828=DIRECTION('ref_axis',(0.,1.,0.));
#12829=DIRECTION('',(0.,1.,0.));
#12830=DIRECTION('',(1.,0.,0.));
#12831=DIRECTION('center_axis',(0.,-1.,0.));
#12832=DIRECTION('ref_axis',(0.,0.,-1.));
#12833=DIRECTION('',(0.,0.,-1.));
#12834=DIRECTION('',(1.,0.,0.));
#12835=DIRECTION('center_axis',(0.,0.,1.));
#12836=DIRECTION('ref_axis',(0.,-1.,0.));
#12837=DIRECTION('',(0.,-1.,0.));
#12838=DIRECTION('',(1.,0.,0.));
#12839=DIRECTION('center_axis',(0.,1.,0.));
#12840=DIRECTION('ref_axis',(0.,0.,1.));
#12841=DIRECTION('',(0.,0.,1.));
#12842=DIRECTION('',(1.,0.,0.));
#12843=DIRECTION('center_axis',(0.,0.,-1.));
#12844=DIRECTION('ref_axis',(0.,1.,0.));
#12845=DIRECTION('',(0.,1.,0.));
#12846=DIRECTION('center_axis',(0.,0.,-1.));
#12847=DIRECTION('ref_axis',(0.,1.,0.));
#12848=DIRECTION('',(0.,1.,0.));
#12849=DIRECTION('',(1.,0.,0.));
#12850=DIRECTION('center_axis',(0.,-1.,0.));
#12851=DIRECTION('ref_axis',(0.,0.,-1.));
#12852=DIRECTION('',(0.,0.,-1.));
#12853=DIRECTION('',(1.,0.,0.));
#12854=DIRECTION('center_axis',(0.,0.,-1.));
#12855=DIRECTION('ref_axis',(0.,1.,0.));
#12856=DIRECTION('',(0.,1.,0.));
#12857=DIRECTION('',(1.,0.,0.));
#12858=DIRECTION('center_axis',(0.,1.,0.));
#12859=DIRECTION('ref_axis',(0.,0.,1.));
#12860=DIRECTION('',(0.,0.,1.));
#12861=DIRECTION('',(1.,0.,0.));
#12862=DIRECTION('center_axis',(0.,0.,-1.));
#12863=DIRECTION('ref_axis',(0.,1.,0.));
#12864=DIRECTION('',(0.,1.,0.));
#12865=DIRECTION('center_axis',(1.,0.,0.));
#12866=DIRECTION('ref_axis',(0.,0.,-1.));
#16250=CARTESIAN_POINT('',(0.,0.,0.));
#16251=CARTESIAN_POINT('Origin',(1.5,-1.9,1.7));
#16252=CARTESIAN_POINT('',(1.56403124237433,-1.7,1.7));
#16253=CARTESIAN_POINT('',(1.43596875762567,-1.7,1.7));
#16254=CARTESIAN_POINT('',(0.75,-1.7,1.7));
#16255=CARTESIAN_POINT('Origin',(1.5,-1.9,1.7));
#16256=CARTESIAN_POINT('Origin',(1.5,-1.9,1.7));
#16257=CARTESIAN_POINT('',(1.56403124237433,-1.7,1.75));
#16258=CARTESIAN_POINT('',(1.56403124237433,-1.7,1.7));
#16259=CARTESIAN_POINT('',(1.29,-1.9,1.75));
#16260=CARTESIAN_POINT('Origin',(1.5,-1.9,1.75));
#16261=CARTESIAN_POINT('',(1.29,-1.9,2.4));
#16262=CARTESIAN_POINT('',(1.29,-1.9,1.7));
#16263=CARTESIAN_POINT('Origin',(1.5,-1.9,2.4));
#16264=CARTESIAN_POINT('',(1.43596875762567,-1.7,1.75));
#16265=CARTESIAN_POINT('Origin',(1.5,-1.9,1.75));
#16266=CARTESIAN_POINT('',(1.43596875762567,-1.7,1.7));
#16267=CARTESIAN_POINT('Origin',(-1.5,1.9,1.7));
#16268=CARTESIAN_POINT('',(-1.56403124237433,1.7,1.7));
#16269=CARTESIAN_POINT('',(-1.43596875762567,1.7,1.7));
#16270=CARTESIAN_POINT('',(-0.75,1.7,1.7));
#16271=CARTESIAN_POINT('Origin',(-1.5,1.9,1.7));
#16272=CARTESIAN_POINT('Origin',(-1.5,1.9,1.7));
#16273=CARTESIAN_POINT('',(-1.56403124237433,1.7,1.75));
#16274=CARTESIAN_POINT('',(-1.56403124237433,1.7,1.7));
#16275=CARTESIAN_POINT('',(-1.71,1.9,1.75));
#16276=CARTESIAN_POINT('Origin',(-1.5,1.9,1.75));
#16277=CARTESIAN_POINT('',(-1.71,1.9,2.4));
#16278=CARTESIAN_POINT('',(-1.71,1.9,1.7));
#16279=CARTESIAN_POINT('Origin',(-1.5,1.9,2.4));
#16280=CARTESIAN_POINT('',(-1.43596875762567,1.7,1.75));
#16281=CARTESIAN_POINT('Origin',(-1.5,1.9,1.75));
#16282=CARTESIAN_POINT('',(-1.43596875762567,1.7,1.7));
#16283=CARTESIAN_POINT('Origin',(-1.5,-1.9,1.7));
#16284=CARTESIAN_POINT('',(-1.43596875762567,-1.7,1.7));
#16285=CARTESIAN_POINT('',(-1.56403124237433,-1.7,1.7));
#16286=CARTESIAN_POINT('',(-0.75,-1.7,1.7));
#16287=CARTESIAN_POINT('Origin',(-1.5,-1.9,1.7));
#16288=CARTESIAN_POINT('Origin',(-1.5,-1.9,1.7));
#16289=CARTESIAN_POINT('',(-1.43596875762567,-1.7,1.75));
#16290=CARTESIAN_POINT('',(-1.43596875762567,-1.7,1.7));
#16291=CARTESIAN_POINT('',(-1.71,-1.9,1.75));
#16292=CARTESIAN_POINT('Origin',(-1.5,-1.9,1.75));
#16293=CARTESIAN_POINT('',(-1.71,-1.9,2.4));
#16294=CARTESIAN_POINT('',(-1.71,-1.9,1.7));
#16295=CARTESIAN_POINT('Origin',(-1.5,-1.9,2.4));
#16296=CARTESIAN_POINT('',(-1.56403124237433,-1.7,1.75));
#16297=CARTESIAN_POINT('Origin',(-1.5,-1.9,1.75));
#16298=CARTESIAN_POINT('',(-1.56403124237433,-1.7,1.7));
#16299=CARTESIAN_POINT('Origin',(1.5,1.9,1.7));
#16300=CARTESIAN_POINT('',(1.43596875762567,1.7,1.7));
#16301=CARTESIAN_POINT('',(1.56403124237433,1.7,1.7));
#16302=CARTESIAN_POINT('',(0.75,1.7,1.7));
#16303=CARTESIAN_POINT('Origin',(1.5,1.9,1.7));
#16304=CARTESIAN_POINT('Origin',(1.5,1.9,1.7));
#16305=CARTESIAN_POINT('',(1.43596875762567,1.7,1.75));
#16306=CARTESIAN_POINT('',(1.43596875762567,1.7,1.7));
#16307=CARTESIAN_POINT('',(1.29,1.9,1.75));
#16308=CARTESIAN_POINT('Origin',(1.5,1.9,1.75));
#16309=CARTESIAN_POINT('',(1.29,1.9,2.4));
#16310=CARTESIAN_POINT('',(1.29,1.9,1.7));
#16311=CARTESIAN_POINT('Origin',(1.5,1.9,2.4));
#16312=CARTESIAN_POINT('',(1.56403124237433,1.7,1.75));
#16313=CARTESIAN_POINT('Origin',(1.5,1.9,1.75));
#16314=CARTESIAN_POINT('',(1.56403124237433,1.7,1.7));
#16315=CARTESIAN_POINT('Origin',(0.,-1.7,1.75));
#16316=CARTESIAN_POINT('',(0.,-1.7,1.75));
#16317=CARTESIAN_POINT('',(-1.97,-1.7,1.75));
#16318=CARTESIAN_POINT('',(0.,-1.7,1.75));
#16319=CARTESIAN_POINT('',(-1.97,-1.7,0.43));
#16320=CARTESIAN_POINT('',(-1.97,-1.7,1.75));
#16321=CARTESIAN_POINT('',(1.97,-1.7,0.43));
#16322=CARTESIAN_POINT('',(0.,-1.7,0.43));
#16323=CARTESIAN_POINT('',(1.97,-1.7,1.75));
#16324=CARTESIAN_POINT('',(1.97,-1.7,1.75));
#16325=CARTESIAN_POINT('',(0.,-1.7,1.75));
#16326=CARTESIAN_POINT('Origin',(0.,1.7,0.43));
#16327=CARTESIAN_POINT('',(0.,1.7,1.75));
#16328=CARTESIAN_POINT('',(1.97,1.7,1.75));
#16329=CARTESIAN_POINT('',(0.,1.7,1.75));
#16330=CARTESIAN_POINT('',(1.97,1.7,0.43));
#16331=CARTESIAN_POINT('',(1.97,1.7,0.43));
#16332=CARTESIAN_POINT('',(-1.97,1.7,0.43));
#16333=CARTESIAN_POINT('',(0.,1.7,0.43));
#16334=CARTESIAN_POINT('',(-1.97,1.7,1.75));
#16335=CARTESIAN_POINT('',(-1.97,1.7,0.43));
#16336=CARTESIAN_POINT('',(0.,1.7,1.75));
#16337=CARTESIAN_POINT('Origin',(-1.97,0.,1.415));
#16338=CARTESIAN_POINT('',(-1.97,-2.35,1.75));
#16339=CARTESIAN_POINT('',(-1.97,-2.35,1.75));
#16340=CARTESIAN_POINT('',(-1.97,-2.35,2.4));
#16341=CARTESIAN_POINT('',(-1.97,-2.35,2.4));
#16342=CARTESIAN_POINT('',(-1.97,2.35,2.4));
#16343=CARTESIAN_POINT('',(-1.97,2.35,2.4));
#16344=CARTESIAN_POINT('',(-1.97,2.35,1.75));
#16345=CARTESIAN_POINT('',(-1.97,2.35,1.75));
#16346=CARTESIAN_POINT('',(-1.97,1.7,1.75));
#16347=CARTESIAN_POINT('',(-1.97,0.78,0.43));
#16348=CARTESIAN_POINT('',(-1.97,0.78,0.43));
#16349=CARTESIAN_POINT('',(-1.97,0.78,1.55));
#16350=CARTESIAN_POINT('',(-1.97,0.78,1.55));
#16351=CARTESIAN_POINT('',(-1.97,-0.78,1.55));
#16352=CARTESIAN_POINT('',(-1.97,-0.78,1.55));
#16353=CARTESIAN_POINT('',(-1.97,-0.78,0.43));
#16354=CARTESIAN_POINT('',(-1.97,-0.78,0.43));
#16355=CARTESIAN_POINT('',(-1.97,-1.7,0.43));
#16356=CARTESIAN_POINT('Origin',(0.,-2.35,1.75));
#16357=CARTESIAN_POINT('',(1.97,-2.35,1.75));
#16358=CARTESIAN_POINT('',(1.97,-2.35,1.75));
#16359=CARTESIAN_POINT('',(0.,-2.35,1.75));
#16360=CARTESIAN_POINT('Origin',(0.,-2.35,2.4));
#16361=CARTESIAN_POINT('',(1.97,-2.35,2.4));
#16362=CARTESIAN_POINT('',(1.97,-2.35,2.4));
#16363=CARTESIAN_POINT('',(0.,-2.35,2.4));
#16364=CARTESIAN_POINT('Origin',(0.,2.35,2.4));
#16365=CARTESIAN_POINT('',(1.97,2.35,2.4));
#16366=CARTESIAN_POINT('',(1.97,2.35,2.4));
#16367=CARTESIAN_POINT('',(0.,2.35,2.4));
#16368=CARTESIAN_POINT('Origin',(0.,2.35,1.75));
#16369=CARTESIAN_POINT('',(1.97,2.35,1.75));
#16370=CARTESIAN_POINT('',(1.97,2.35,1.75));
#16371=CARTESIAN_POINT('',(0.,2.35,1.75));
#16372=CARTESIAN_POINT('Origin',(0.,1.7,1.75));
#16373=CARTESIAN_POINT('',(1.97,1.7,1.75));
#16374=CARTESIAN_POINT('Origin',(0.,0.78,0.43));
#16375=CARTESIAN_POINT('',(1.97,0.78,0.43));
#16376=CARTESIAN_POINT('',(1.97,0.78,0.43));
#16377=CARTESIAN_POINT('',(0.,0.78,0.43));
#16378=CARTESIAN_POINT('Origin',(0.,0.78,1.55));
#16379=CARTESIAN_POINT('',(1.97,0.78,1.55));
#16380=CARTESIAN_POINT('',(1.97,0.78,1.55));
#16381=CARTESIAN_POINT('',(0.,0.78,1.55));
#16382=CARTESIAN_POINT('Origin',(0.,-0.78,1.55));
#16383=CARTESIAN_POINT('',(1.97,-0.78,1.55));
#16384=CARTESIAN_POINT('',(1.97,-0.78,1.55));
#16385=CARTESIAN_POINT('',(0.,-0.78,1.55));
#16386=CARTESIAN_POINT('Origin',(0.,-0.78,0.43));
#16387=CARTESIAN_POINT('',(1.97,-0.78,0.43));
#16388=CARTESIAN_POINT('',(1.97,-0.78,0.43));
#16389=CARTESIAN_POINT('',(0.,-0.78,0.43));
#16390=CARTESIAN_POINT('Origin',(0.,-1.7,0.43));
#16391=CARTESIAN_POINT('',(1.97,-1.7,0.43));
#16392=CARTESIAN_POINT('Origin',(1.97,0.,1.415));
#16845=UNCERTAINTY_MEASURE_WITH_UNIT(LENGTH_MEASURE(0.001),#16912,
'DISTANCE_ACCURACY_VALUE',
'Maximum model space distance between geometric entities at asserted c
onnectivities');
#16852=UNCERTAINTY_MEASURE_WITH_UNIT(LENGTH_MEASURE(0.001),#16912,
'DISTANCE_ACCURACY_VALUE',
'Maximum model space distance between geometric entities at asserted c
onnectivities');
#16904=(
GEOMETRIC_REPRESENTATION_CONTEXT(3)
GLOBAL_UNCERTAINTY_ASSIGNED_CONTEXT((#16845))
GLOBAL_UNIT_ASSIGNED_CONTEXT((#16912,#16914,#16915))
REPRESENTATION_CONTEXT('','3D')
);
#16911=(
GEOMETRIC_REPRESENTATION_CONTEXT(3)
GLOBAL_UNCERTAINTY_ASSIGNED_CONTEXT((#16852))
GLOBAL_UNIT_ASSIGNED_CONTEXT((#16912,#16914,#16915))
REPRESENTATION_CONTEXT('','3D')
);
#16912=(
LENGTH_UNIT()
NAMED_UNIT(*)
SI_UNIT(.CENTI.,.METRE.)
);
#16914=(
NAMED_UNIT(*)
PLANE_ANGLE_UNIT()
SI_UNIT($,.RADIAN.)
);
#16915=(
NAMED_UNIT(*)
SI_UNIT($,.STERADIAN.)
SOLID_ANGLE_UNIT()
);
#16967=SHAPE_DEFINITION_REPRESENTATION(#17039,#17175);
#17039=PRODUCT_DEFINITION_SHAPE('',$,#17234);
#17175=SHAPE_REPRESENTATION('',(#10342),#16904);
#17182=PRODUCT_DEFINITION_CONTEXT('part definition',#17358,'design');
#17234=PRODUCT_DEFINITION('Block','Block',#17292,#17182);
#17292=PRODUCT_DEFINITION_FORMATION('',$,#17411);
#17358=APPLICATION_CONTEXT(
'Core Data for Automotive Mechanical Design Process');
#17359=PRODUCT_CONTEXT('part definition',#17358,'mechanical');
#17411=PRODUCT('Block','Block','Block',(#17359));
#17460=COLOUR_RGB('Dark Blue',0.08,0.2,0.34);
#17461=FILL_AREA_STYLE_COLOUR('',#17460);
#17462=FILL_AREA_STYLE('',(#17461));
#17463=SURFACE_STYLE_FILL_AREA(#17462);
#17464=SURFACE_SIDE_STYLE('',(#17463));
#17465=SURFACE_STYLE_USAGE(.BOTH.,#17464);
#17466=PRESENTATION_STYLE_ASSIGNMENT((#17465));
ENDSEC;
END-ISO-10303-21;
